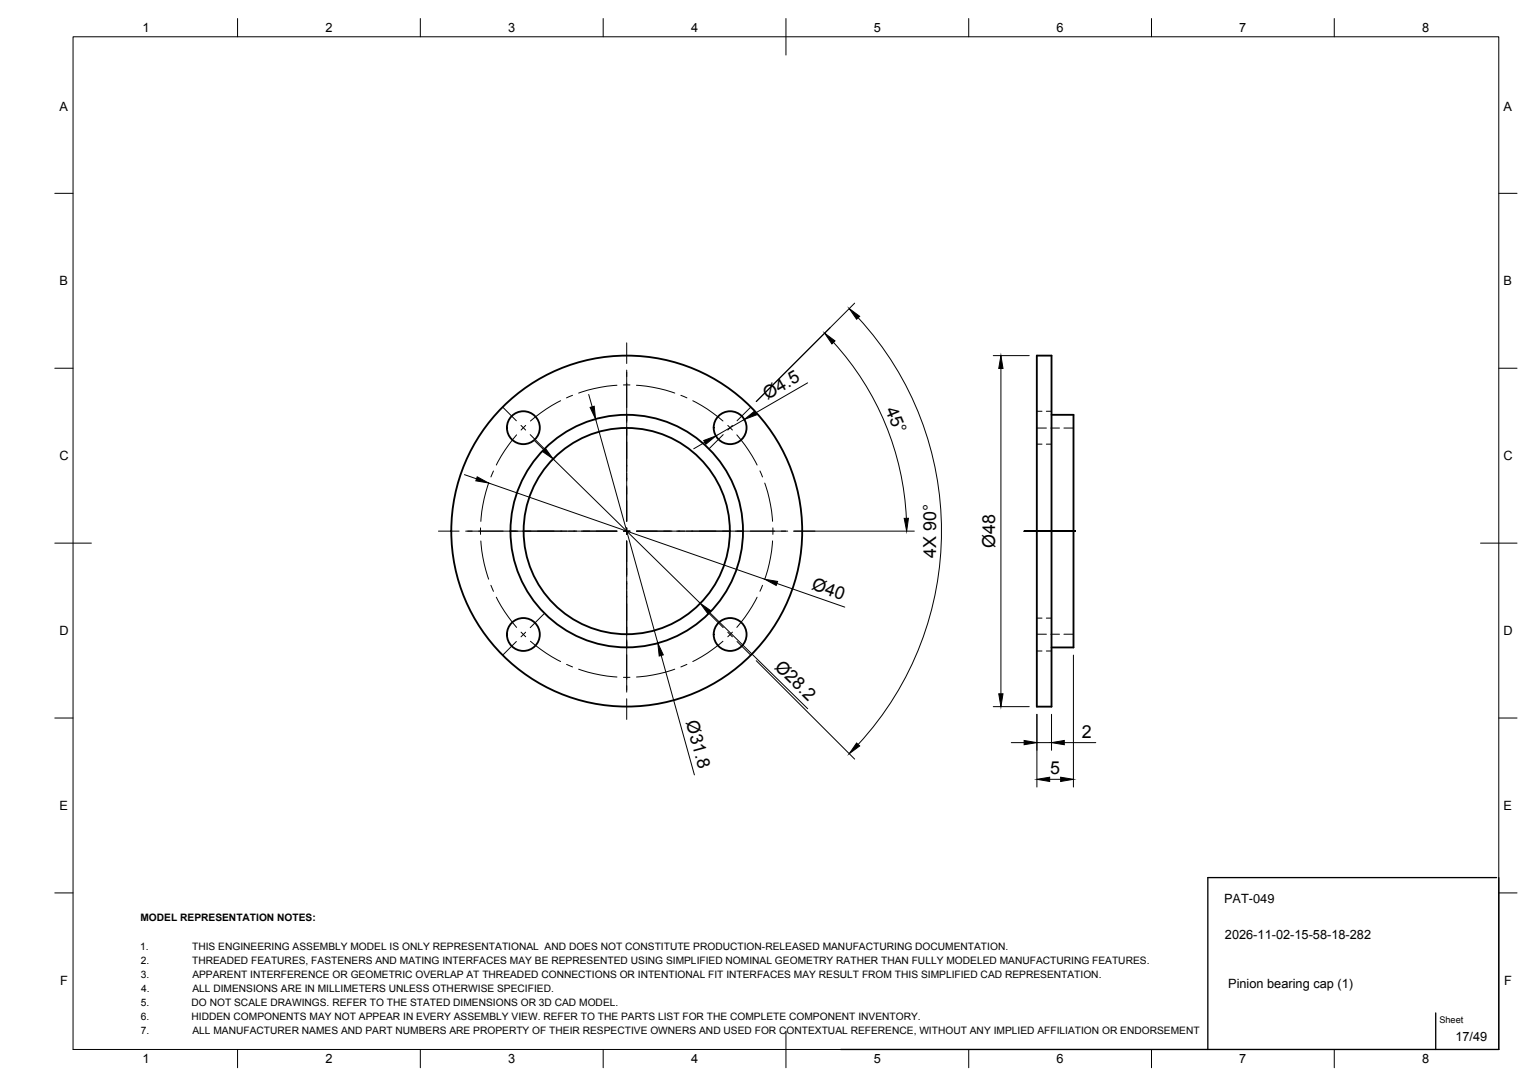
ISO-10303-21;
HEADER;
/* Generated by software containing ST-Developer
 * from STEP Tools, Inc. (www.steptools.com) 
 */

FILE_DESCRIPTION(
/* description */ ('Hand drill press frame (manual)'),
/* implementation_level */ '2;1');

FILE_NAME(
/* name */ 'Pinion bearing cap (1).step',
/* time_stamp */ '2026-10-28T03:25:28-07:00',
/* author */ (''),
/* organization */ (''),
/* preprocessor_version */ 'ST-DEVELOPER v20.2',
/* originating_system */ 'Autodesk Translation Framework v15.17.0.0',
/* authorisation */ '');

FILE_SCHEMA (('AUTOMOTIVE_DESIGN { 1 0 10303 214 3 1 1 }'));
ENDSEC;

DATA;
#10=MECHANICAL_DESIGN_GEOMETRIC_PRESENTATION_REPRESENTATION('',(#631),#33299);
#541=SHAPE_REPRESENTATION_RELATIONSHIP('SRR','None',#33500,#586);
#586=ADVANCED_BREP_SHAPE_REPRESENTATION('',(#683),#33262);
#631=STYLED_ITEM('',(#33814),#683);
#683=MANIFOLD_SOLID_BREP('Body1',#12649);
#789=FACE_BOUND('',#2269,.T.);
#790=FACE_BOUND('',#2273,.T.);
#791=FACE_BOUND('',#2274,.T.);
#792=FACE_BOUND('',#2275,.T.);
#793=FACE_BOUND('',#2276,.T.);
#794=FACE_BOUND('',#2277,.T.);
#795=FACE_BOUND('',#2279,.T.);
#796=FACE_BOUND('',#2280,.T.);
#797=FACE_BOUND('',#2281,.T.);
#798=FACE_BOUND('',#2282,.T.);
#799=FACE_BOUND('',#2283,.T.);
#996=PLANE('',#13504);
#997=PLANE('',#13511);
#998=PLANE('',#13512);
#1505=FACE_OUTER_BOUND('',#2263,.T.);
#1506=FACE_OUTER_BOUND('',#2264,.T.);
#1507=FACE_OUTER_BOUND('',#2265,.T.);
#1508=FACE_OUTER_BOUND('',#2266,.T.);
#1509=FACE_OUTER_BOUND('',#2267,.T.);
#1510=FACE_OUTER_BOUND('',#2268,.T.);
#1511=FACE_OUTER_BOUND('',#2270,.T.);
#1512=FACE_OUTER_BOUND('',#2271,.T.);
#1513=FACE_OUTER_BOUND('',#2272,.T.);
#1514=FACE_OUTER_BOUND('',#2278,.T.);
#2263=EDGE_LOOP('',(#9221,#9222,#9223,#9224));
#2264=EDGE_LOOP('',(#9225,#9226,#9227,#9228));
#2265=EDGE_LOOP('',(#9229,#9230,#9231,#9232));
#2266=EDGE_LOOP('',(#9233,#9234,#9235,#9236));
#2267=EDGE_LOOP('',(#9237,#9238,#9239,#9240));
#2268=EDGE_LOOP('',(#9241));
#2269=EDGE_LOOP('',(#9242));
#2270=EDGE_LOOP('',(#9243,#9244,#9245,#9246));
#2271=EDGE_LOOP('',(#9247,#9248,#9249,#9250));
#2272=EDGE_LOOP('',(#9251));
#2273=EDGE_LOOP('',(#9252));
#2274=EDGE_LOOP('',(#9253));
#2275=EDGE_LOOP('',(#9254));
#2276=EDGE_LOOP('',(#9255));
#2277=EDGE_LOOP('',(#9256));
#2278=EDGE_LOOP('',(#9257));
#2279=EDGE_LOOP('',(#9258));
#2280=EDGE_LOOP('',(#9259));
#2281=EDGE_LOOP('',(#9260));
#2282=EDGE_LOOP('',(#9261));
#2283=EDGE_LOOP('',(#9262));
#3149=LINE('',#18925,#4314);
#3150=LINE('',#18931,#4315);
#3151=LINE('',#18937,#4316);
#3152=LINE('',#18943,#4317);
#3153=LINE('',#18949,#4318);
#3154=LINE('',#18957,#4319);
#3155=LINE('',#18962,#4320);
#4314=VECTOR('',#15238,0.225);
#4315=VECTOR('',#15245,0.225);
#4316=VECTOR('',#15252,0.225);
#4317=VECTOR('',#15259,0.225);
#4318=VECTOR('',#15266,1.59);
#4319=VECTOR('',#15277,1.41);
#4320=VECTOR('',#15282,2.4);
#5334=CIRCLE('',#13490,0.225);
#5335=CIRCLE('',#13491,0.225);
#5336=CIRCLE('',#13493,0.225);
#5337=CIRCLE('',#13494,0.225);
#5338=CIRCLE('',#13496,0.225);
#5339=CIRCLE('',#13497,0.225);
#5340=CIRCLE('',#13499,0.225);
#5341=CIRCLE('',#13500,0.225);
#5342=CIRCLE('',#13502,1.59);
#5343=CIRCLE('',#13503,1.59);
#5344=CIRCLE('',#13505,1.41);
#5345=CIRCLE('',#13507,1.41);
#5346=CIRCLE('',#13509,2.4);
#5347=CIRCLE('',#13510,2.4);
#5880=VERTEX_POINT('',#18922);
#5881=VERTEX_POINT('',#18924);
#5882=VERTEX_POINT('',#18928);
#5883=VERTEX_POINT('',#18930);
#5884=VERTEX_POINT('',#18934);
#5885=VERTEX_POINT('',#18936);
#5886=VERTEX_POINT('',#18940);
#5887=VERTEX_POINT('',#18942);
#5888=VERTEX_POINT('',#18946);
#5889=VERTEX_POINT('',#18948);
#5890=VERTEX_POINT('',#18952);
#5891=VERTEX_POINT('',#18955);
#5892=VERTEX_POINT('',#18959);
#5893=VERTEX_POINT('',#18961);
#7139=EDGE_CURVE('',#5880,#5880,#5334,.T.);
#7140=EDGE_CURVE('',#5880,#5881,#3149,.T.);
#7141=EDGE_CURVE('',#5881,#5881,#5335,.T.);
#7142=EDGE_CURVE('',#5882,#5882,#5336,.T.);
#7143=EDGE_CURVE('',#5882,#5883,#3150,.T.);
#7144=EDGE_CURVE('',#5883,#5883,#5337,.T.);
#7145=EDGE_CURVE('',#5884,#5884,#5338,.T.);
#7146=EDGE_CURVE('',#5884,#5885,#3151,.T.);
#7147=EDGE_CURVE('',#5885,#5885,#5339,.T.);
#7148=EDGE_CURVE('',#5886,#5886,#5340,.T.);
#7149=EDGE_CURVE('',#5886,#5887,#3152,.T.);
#7150=EDGE_CURVE('',#5887,#5887,#5341,.T.);
#7151=EDGE_CURVE('',#5888,#5888,#5342,.T.);
#7152=EDGE_CURVE('',#5888,#5889,#3153,.T.);
#7153=EDGE_CURVE('',#5889,#5889,#5343,.T.);
#7154=EDGE_CURVE('',#5890,#5890,#5344,.T.);
#7155=EDGE_CURVE('',#5891,#5891,#5345,.T.);
#7156=EDGE_CURVE('',#5891,#5890,#3154,.T.);
#7157=EDGE_CURVE('',#5892,#5892,#5346,.T.);
#7158=EDGE_CURVE('',#5892,#5893,#3155,.T.);
#7159=EDGE_CURVE('',#5893,#5893,#5347,.T.);
#9221=ORIENTED_EDGE('',*,*,#7139,.F.);
#9222=ORIENTED_EDGE('',*,*,#7140,.T.);
#9223=ORIENTED_EDGE('',*,*,#7141,.F.);
#9224=ORIENTED_EDGE('',*,*,#7140,.F.);
#9225=ORIENTED_EDGE('',*,*,#7142,.F.);
#9226=ORIENTED_EDGE('',*,*,#7143,.T.);
#9227=ORIENTED_EDGE('',*,*,#7144,.F.);
#9228=ORIENTED_EDGE('',*,*,#7143,.F.);
#9229=ORIENTED_EDGE('',*,*,#7145,.F.);
#9230=ORIENTED_EDGE('',*,*,#7146,.T.);
#9231=ORIENTED_EDGE('',*,*,#7147,.F.);
#9232=ORIENTED_EDGE('',*,*,#7146,.F.);
#9233=ORIENTED_EDGE('',*,*,#7148,.F.);
#9234=ORIENTED_EDGE('',*,*,#7149,.T.);
#9235=ORIENTED_EDGE('',*,*,#7150,.F.);
#9236=ORIENTED_EDGE('',*,*,#7149,.F.);
#9237=ORIENTED_EDGE('',*,*,#7151,.F.);
#9238=ORIENTED_EDGE('',*,*,#7152,.T.);
#9239=ORIENTED_EDGE('',*,*,#7153,.T.);
#9240=ORIENTED_EDGE('',*,*,#7152,.F.);
#9241=ORIENTED_EDGE('',*,*,#7153,.F.);
#9242=ORIENTED_EDGE('',*,*,#7154,.F.);
#9243=ORIENTED_EDGE('',*,*,#7155,.F.);
#9244=ORIENTED_EDGE('',*,*,#7156,.T.);
#9245=ORIENTED_EDGE('',*,*,#7154,.T.);
#9246=ORIENTED_EDGE('',*,*,#7156,.F.);
#9247=ORIENTED_EDGE('',*,*,#7157,.F.);
#9248=ORIENTED_EDGE('',*,*,#7158,.T.);
#9249=ORIENTED_EDGE('',*,*,#7159,.T.);
#9250=ORIENTED_EDGE('',*,*,#7158,.F.);
#9251=ORIENTED_EDGE('',*,*,#7157,.T.);
#9252=ORIENTED_EDGE('',*,*,#7155,.T.);
#9253=ORIENTED_EDGE('',*,*,#7150,.T.);
#9254=ORIENTED_EDGE('',*,*,#7147,.T.);
#9255=ORIENTED_EDGE('',*,*,#7144,.T.);
#9256=ORIENTED_EDGE('',*,*,#7141,.T.);
#9257=ORIENTED_EDGE('',*,*,#7159,.F.);
#9258=ORIENTED_EDGE('',*,*,#7151,.T.);
#9259=ORIENTED_EDGE('',*,*,#7148,.T.);
#9260=ORIENTED_EDGE('',*,*,#7145,.T.);
#9261=ORIENTED_EDGE('',*,*,#7142,.T.);
#9262=ORIENTED_EDGE('',*,*,#7139,.T.);
#11842=CYLINDRICAL_SURFACE('',#13489,0.225);
#11843=CYLINDRICAL_SURFACE('',#13492,0.225);
#11844=CYLINDRICAL_SURFACE('',#13495,0.225);
#11845=CYLINDRICAL_SURFACE('',#13498,0.225);
#11846=CYLINDRICAL_SURFACE('',#13501,1.59);
#11847=CYLINDRICAL_SURFACE('',#13506,1.41);
#11848=CYLINDRICAL_SURFACE('',#13508,2.4);
#12114=ADVANCED_FACE('',(#1505),#11842,.F.);
#12115=ADVANCED_FACE('',(#1506),#11843,.F.);
#12116=ADVANCED_FACE('',(#1507),#11844,.F.);
#12117=ADVANCED_FACE('',(#1508),#11845,.F.);
#12118=ADVANCED_FACE('',(#1509),#11846,.T.);
#12119=ADVANCED_FACE('',(#1510,#789),#996,.F.);
#12120=ADVANCED_FACE('',(#1511),#11847,.F.);
#12121=ADVANCED_FACE('',(#1512),#11848,.T.);
#12122=ADVANCED_FACE('',(#1513,#790,#791,#792,#793,#794),#997,.T.);
#12123=ADVANCED_FACE('',(#1514,#795,#796,#797,#798,#799),#998,.F.);
#12649=CLOSED_SHELL('',(#12114,#12115,#12116,#12117,#12118,#12119,#12120,
#12121,#12122,#12123));
#13488=AXIS2_PLACEMENT_3D('',#18920,#15232,#15233);
#13489=AXIS2_PLACEMENT_3D('',#18921,#15234,#15235);
#13490=AXIS2_PLACEMENT_3D('',#18923,#15236,#15237);
#13491=AXIS2_PLACEMENT_3D('',#18926,#15239,#15240);
#13492=AXIS2_PLACEMENT_3D('',#18927,#15241,#15242);
#13493=AXIS2_PLACEMENT_3D('',#18929,#15243,#15244);
#13494=AXIS2_PLACEMENT_3D('',#18932,#15246,#15247);
#13495=AXIS2_PLACEMENT_3D('',#18933,#15248,#15249);
#13496=AXIS2_PLACEMENT_3D('',#18935,#15250,#15251);
#13497=AXIS2_PLACEMENT_3D('',#18938,#15253,#15254);
#13498=AXIS2_PLACEMENT_3D('',#18939,#15255,#15256);
#13499=AXIS2_PLACEMENT_3D('',#18941,#15257,#15258);
#13500=AXIS2_PLACEMENT_3D('',#18944,#15260,#15261);
#13501=AXIS2_PLACEMENT_3D('',#18945,#15262,#15263);
#13502=AXIS2_PLACEMENT_3D('',#18947,#15264,#15265);
#13503=AXIS2_PLACEMENT_3D('',#18950,#15267,#15268);
#13504=AXIS2_PLACEMENT_3D('',#18951,#15269,#15270);
#13505=AXIS2_PLACEMENT_3D('',#18953,#15271,#15272);
#13506=AXIS2_PLACEMENT_3D('',#18954,#15273,#15274);
#13507=AXIS2_PLACEMENT_3D('',#18956,#15275,#15276);
#13508=AXIS2_PLACEMENT_3D('',#18958,#15278,#15279);
#13509=AXIS2_PLACEMENT_3D('',#18960,#15280,#15281);
#13510=AXIS2_PLACEMENT_3D('',#18963,#15283,#15284);
#13511=AXIS2_PLACEMENT_3D('',#18964,#15285,#15286);
#13512=AXIS2_PLACEMENT_3D('',#18965,#15287,#15288);
#15232=DIRECTION('axis',(0.,0.,1.));
#15233=DIRECTION('refdir',(1.,0.,0.));
#15234=DIRECTION('center_axis',(0.,1.,0.));
#15235=DIRECTION('ref_axis',(1.,0.,0.));
#15236=DIRECTION('center_axis',(0.,1.,0.));
#15237=DIRECTION('ref_axis',(1.,0.,0.));
#15238=DIRECTION('',(0.,1.,0.));
#15239=DIRECTION('center_axis',(0.,-1.,0.));
#15240=DIRECTION('ref_axis',(1.,0.,0.));
#15241=DIRECTION('center_axis',(0.,1.,0.));
#15242=DIRECTION('ref_axis',(1.,0.,0.));
#15243=DIRECTION('center_axis',(0.,1.,0.));
#15244=DIRECTION('ref_axis',(1.,0.,0.));
#15245=DIRECTION('',(0.,1.,0.));
#15246=DIRECTION('center_axis',(0.,-1.,0.));
#15247=DIRECTION('ref_axis',(1.,0.,0.));
#15248=DIRECTION('center_axis',(0.,1.,0.));
#15249=DIRECTION('ref_axis',(1.,0.,0.));
#15250=DIRECTION('center_axis',(0.,1.,0.));
#15251=DIRECTION('ref_axis',(1.,0.,0.));
#15252=DIRECTION('',(0.,1.,0.));
#15253=DIRECTION('center_axis',(0.,-1.,0.));
#15254=DIRECTION('ref_axis',(1.,0.,0.));
#15255=DIRECTION('center_axis',(0.,1.,0.));
#15256=DIRECTION('ref_axis',(1.,0.,0.));
#15257=DIRECTION('center_axis',(0.,1.,0.));
#15258=DIRECTION('ref_axis',(1.,0.,0.));
#15259=DIRECTION('',(0.,1.,0.));
#15260=DIRECTION('center_axis',(0.,-1.,0.));
#15261=DIRECTION('ref_axis',(1.,0.,0.));
#15262=DIRECTION('center_axis',(0.,1.,0.));
#15263=DIRECTION('ref_axis',(1.,0.,0.));
#15264=DIRECTION('center_axis',(0.,1.,0.));
#15265=DIRECTION('ref_axis',(1.,0.,0.));
#15266=DIRECTION('',(0.,-1.,0.));
#15267=DIRECTION('center_axis',(0.,1.,0.));
#15268=DIRECTION('ref_axis',(1.,0.,0.));
#15269=DIRECTION('center_axis',(0.,1.,0.));
#15270=DIRECTION('ref_axis',(1.,0.,0.));
#15271=DIRECTION('center_axis',(0.,-1.,0.));
#15272=DIRECTION('ref_axis',(1.,0.,0.));
#15273=DIRECTION('center_axis',(0.,1.,0.));
#15274=DIRECTION('ref_axis',(1.,0.,0.));
#15275=DIRECTION('center_axis',(0.,-1.,0.));
#15276=DIRECTION('ref_axis',(1.,0.,0.));
#15277=DIRECTION('',(0.,-1.,0.));
#15278=DIRECTION('center_axis',(0.,1.,0.));
#15279=DIRECTION('ref_axis',(1.,0.,0.));
#15280=DIRECTION('center_axis',(0.,1.,0.));
#15281=DIRECTION('ref_axis',(1.,0.,0.));
#15282=DIRECTION('',(0.,-1.,0.));
#15283=DIRECTION('center_axis',(0.,1.,0.));
#15284=DIRECTION('ref_axis',(1.,0.,0.));
#15285=DIRECTION('center_axis',(0.,1.,0.));
#15286=DIRECTION('ref_axis',(1.,0.,0.));
#15287=DIRECTION('center_axis',(0.,1.,0.));
#15288=DIRECTION('ref_axis',(1.,0.,0.));
#18920=CARTESIAN_POINT('',(0.,0.,0.));
#18921=CARTESIAN_POINT('Origin',(-4.66421356237309,-2.3,18.5857864376269));
#18922=CARTESIAN_POINT('',(-4.88921356237309,-2.2,18.5857864376269));
#18923=CARTESIAN_POINT('Origin',(-4.66421356237309,-2.2,18.5857864376269));
#18924=CARTESIAN_POINT('',(-4.88921356237309,-2.,18.5857864376269));
#18925=CARTESIAN_POINT('',(-4.88921356237309,-2.3,18.5857864376269));
#18926=CARTESIAN_POINT('Origin',(-4.66421356237309,-2.,18.5857864376269));
#18927=CARTESIAN_POINT('Origin',(-4.66421356237309,-2.3,21.4142135623731));
#18928=CARTESIAN_POINT('',(-4.88921356237309,-2.2,21.4142135623731));
#18929=CARTESIAN_POINT('Origin',(-4.66421356237309,-2.2,21.4142135623731));
#18930=CARTESIAN_POINT('',(-4.88921356237309,-2.,21.4142135623731));
#18931=CARTESIAN_POINT('',(-4.88921356237309,-2.3,21.4142135623731));
#18932=CARTESIAN_POINT('Origin',(-4.66421356237309,-2.,21.4142135623731));
#18933=CARTESIAN_POINT('Origin',(-1.8357864376269,-2.3,21.4142135623731));
#18934=CARTESIAN_POINT('',(-2.0607864376269,-2.2,21.4142135623731));
#18935=CARTESIAN_POINT('Origin',(-1.8357864376269,-2.2,21.4142135623731));
#18936=CARTESIAN_POINT('',(-2.0607864376269,-2.,21.4142135623731));
#18937=CARTESIAN_POINT('',(-2.0607864376269,-2.3,21.4142135623731));
#18938=CARTESIAN_POINT('Origin',(-1.8357864376269,-2.,21.4142135623731));
#18939=CARTESIAN_POINT('Origin',(-1.83578643762691,-2.3,18.5857864376269));
#18940=CARTESIAN_POINT('',(-2.06078643762691,-2.2,18.5857864376269));
#18941=CARTESIAN_POINT('Origin',(-1.83578643762691,-2.2,18.5857864376269));
#18942=CARTESIAN_POINT('',(-2.06078643762691,-2.,18.5857864376269));
#18943=CARTESIAN_POINT('',(-2.06078643762691,-2.3,18.5857864376269));
#18944=CARTESIAN_POINT('Origin',(-1.83578643762691,-2.,18.5857864376269));
#18945=CARTESIAN_POINT('Origin',(-3.25,-2.5,20.));
#18946=CARTESIAN_POINT('',(-4.84,-2.2,20.));
#18947=CARTESIAN_POINT('Origin',(-3.25,-2.2,20.));
#18948=CARTESIAN_POINT('',(-4.84,-2.5,20.));
#18949=CARTESIAN_POINT('',(-4.84,-2.5,20.));
#18950=CARTESIAN_POINT('Origin',(-3.25,-2.5,20.));
#18951=CARTESIAN_POINT('Origin',(-3.25,-2.5,20.));
#18952=CARTESIAN_POINT('',(-4.66,-2.5,20.));
#18953=CARTESIAN_POINT('Origin',(-3.25,-2.5,20.));
#18954=CARTESIAN_POINT('Origin',(-3.25,-2.2,20.));
#18955=CARTESIAN_POINT('',(-4.66,-2.,20.));
#18956=CARTESIAN_POINT('Origin',(-3.25,-2.,20.));
#18957=CARTESIAN_POINT('',(-4.66,-2.2,20.));
#18958=CARTESIAN_POINT('Origin',(-3.25,-2.2,20.));
#18959=CARTESIAN_POINT('',(-5.65,-2.,20.));
#18960=CARTESIAN_POINT('Origin',(-3.25,-2.,20.));
#18961=CARTESIAN_POINT('',(-5.65,-2.2,20.));
#18962=CARTESIAN_POINT('',(-5.65,-2.2,20.));
#18963=CARTESIAN_POINT('Origin',(-3.25,-2.2,20.));
#18964=CARTESIAN_POINT('Origin',(-3.25,-2.,20.));
#18965=CARTESIAN_POINT('Origin',(-3.25,-2.2,20.));
#33210=UNCERTAINTY_MEASURE_WITH_UNIT(LENGTH_MEASURE(0.001),#33300,
'DISTANCE_ACCURACY_VALUE',
'Maximum model space distance between geometric entities at asserted c
onnectivities');
#33247=UNCERTAINTY_MEASURE_WITH_UNIT(LENGTH_MEASURE(0.001),#33300,
'DISTANCE_ACCURACY_VALUE',
'Maximum model space distance between geometric entities at asserted c
onnectivities');
#33262=(
GEOMETRIC_REPRESENTATION_CONTEXT(3)
GLOBAL_UNCERTAINTY_ASSIGNED_CONTEXT((#33210))
GLOBAL_UNIT_ASSIGNED_CONTEXT((#33300,#33302,#33303))
REPRESENTATION_CONTEXT('','3D')
);
#33299=(
GEOMETRIC_REPRESENTATION_CONTEXT(3)
GLOBAL_UNCERTAINTY_ASSIGNED_CONTEXT((#33247))
GLOBAL_UNIT_ASSIGNED_CONTEXT((#33300,#33302,#33303))
REPRESENTATION_CONTEXT('','3D')
);
#33300=(
LENGTH_UNIT()
NAMED_UNIT(*)
SI_UNIT(.CENTI.,.METRE.)
);
#33302=(
NAMED_UNIT(*)
PLANE_ANGLE_UNIT()
SI_UNIT($,.RADIAN.)
);
#33303=(
NAMED_UNIT(*)
SI_UNIT($,.STERADIAN.)
SOLID_ANGLE_UNIT()
);
#33318=SHAPE_DEFINITION_REPRESENTATION(#33369,#33500);
#33369=PRODUCT_DEFINITION_SHAPE('',$,#33552);
#33500=SHAPE_REPRESENTATION('',(#13488),#33262);
#33537=PRODUCT_DEFINITION_CONTEXT('part definition',#33692,'design');
#33552=PRODUCT_DEFINITION('Pinion bearing cap (1)',
'Pinion bearing cap (1)',#33603,#33537);
#33603=PRODUCT_DEFINITION_FORMATION('',$,#33708);
#33692=APPLICATION_CONTEXT(
'Core Data for Automotive Mechanical Design Process');
#33693=PRODUCT_CONTEXT('part definition',#33692,'mechanical');
#33708=PRODUCT('Pinion bearing cap (1)','Pinion bearing cap (1)',
'Pinion bearing cap (1)',(#33693));
#33808=COLOUR_RGB('Grey',0.48,0.52,0.57);
#33809=FILL_AREA_STYLE_COLOUR('',#33808);
#33810=FILL_AREA_STYLE('',(#33809));
#33811=SURFACE_STYLE_FILL_AREA(#33810);
#33812=SURFACE_SIDE_STYLE('',(#33811));
#33813=SURFACE_STYLE_USAGE(.BOTH.,#33812);
#33814=PRESENTATION_STYLE_ASSIGNMENT((#33813));
ENDSEC;
END-ISO-10303-21;
